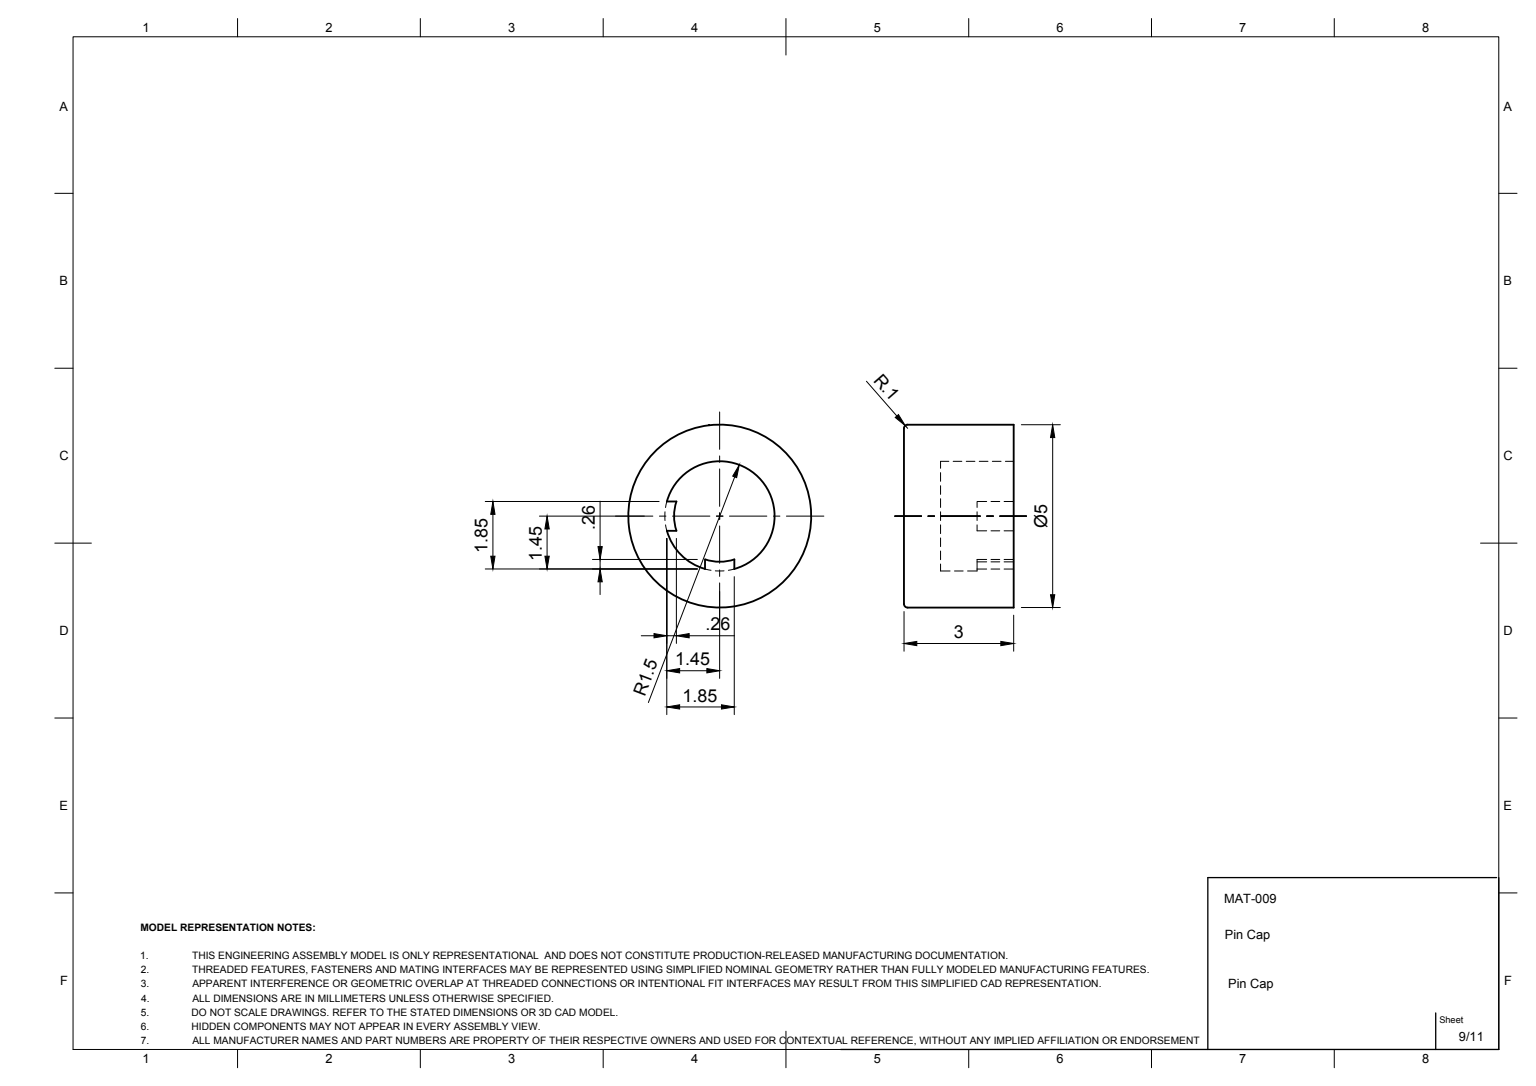
ISO-10303-21;
HEADER;
/* Generated by software containing ST-Developer
 * from STEP Tools, Inc. (www.steptools.com) 
 */

FILE_DESCRIPTION(
/* description */ ('STEP AP214'),
/* implementation_level */ '2;1');

FILE_NAME(
/* name */ 'Pin Cap.step',
/* time_stamp */ '2026-11-14T05:43:09-08:00',
/* author */ (''),
/* organization */ (''),
/* preprocessor_version */ 'ST-DEVELOPER v20.2',
/* originating_system */ 'Autodesk Translation Framework v15.17.0.0',
/* authorisation */ '');

FILE_SCHEMA (('AUTOMOTIVE_DESIGN { 1 0 10303 214 3 1 1 }'));
ENDSEC;

DATA;
#10=MECHANICAL_DESIGN_GEOMETRIC_PRESENTATION_REPRESENTATION('',(#154),#11933);
#127=TOROIDAL_SURFACE('',#7592,2.4,0.1);
#136=SHAPE_REPRESENTATION_RELATIONSHIP('SRR','None',#11996,#145);
#145=ADVANCED_BREP_SHAPE_REPRESENTATION('',(#163),#11932);
#154=STYLED_ITEM('',(#12043),#163);
#163=MANIFOLD_SOLID_BREP('Body1',#6651);
#208=FACE_BOUND('',#1064,.T.);
#310=PLANE('',#7609);
#311=PLANE('',#7611);
#312=PLANE('',#7612);
#313=PLANE('',#7615);
#314=PLANE('',#7616);
#315=PLANE('',#7617);
#316=PLANE('',#7618);
#317=PLANE('',#7619);
#318=PLANE('',#7620);
#659=FACE_OUTER_BOUND('',#1057,.T.);
#660=FACE_OUTER_BOUND('',#1058,.T.);
#661=FACE_OUTER_BOUND('',#1059,.T.);
#662=FACE_OUTER_BOUND('',#1060,.T.);
#663=FACE_OUTER_BOUND('',#1061,.T.);
#664=FACE_OUTER_BOUND('',#1062,.T.);
#665=FACE_OUTER_BOUND('',#1063,.T.);
#666=FACE_OUTER_BOUND('',#1065,.T.);
#667=FACE_OUTER_BOUND('',#1066,.T.);
#668=FACE_OUTER_BOUND('',#1067,.T.);
#669=FACE_OUTER_BOUND('',#1068,.T.);
#670=FACE_OUTER_BOUND('',#1069,.T.);
#671=FACE_OUTER_BOUND('',#1070,.T.);
#672=FACE_OUTER_BOUND('',#1071,.T.);
#1057=EDGE_LOOP('',(#5980,#5981,#5982,#5983,#5984));
#1058=EDGE_LOOP('',(#5985,#5986,#5987,#5988));
#1059=EDGE_LOOP('',(#5989,#5990,#5991,#5992,#5993));
#1060=EDGE_LOOP('',(#5994,#5995,#5996,#5997,#5998,#5999,#6000,#6001,#6002,
#6003,#6004,#6005));
#1061=EDGE_LOOP('',(#6006,#6007,#6008,#6009));
#1062=EDGE_LOOP('',(#6010,#6011,#6012,#6013));
#1063=EDGE_LOOP('',(#6014));
#1064=EDGE_LOOP('',(#6015,#6016,#6017,#6018,#6019,#6020,#6021,#6022,#6023));
#1065=EDGE_LOOP('',(#6024,#6025,#6026,#6027));
#1066=EDGE_LOOP('',(#6028,#6029,#6030,#6031));
#1067=EDGE_LOOP('',(#6032,#6033,#6034,#6035));
#1068=EDGE_LOOP('',(#6036,#6037,#6038,#6039));
#1069=EDGE_LOOP('',(#6040,#6041,#6042,#6043));
#1070=EDGE_LOOP('',(#6044));
#1071=EDGE_LOOP('',(#6045));
#1516=LINE('',#11827,#1978);
#1517=LINE('',#11830,#1979);
#1518=LINE('',#11833,#1980);
#1519=LINE('',#11840,#1981);
#1520=LINE('',#11844,#1982);
#1521=LINE('',#11849,#1983);
#1522=LINE('',#11853,#1984);
#1523=LINE('',#11856,#1985);
#1524=LINE('',#11859,#1986);
#1525=LINE('',#11862,#1987);
#1526=LINE('',#11864,#1988);
#1527=LINE('',#11865,#1989);
#1528=LINE('',#11868,#1990);
#1529=LINE('',#11871,#1991);
#1530=LINE('',#11872,#1992);
#1531=LINE('',#11873,#1993);
#1532=LINE('',#11875,#1994);
#1533=LINE('',#11876,#1995);
#1978=VECTOR('',#9788,1000.);
#1979=VECTOR('',#9791,1000.);
#1980=VECTOR('',#9794,2.5);
#1981=VECTOR('',#9801,1000.);
#1982=VECTOR('',#9804,1.5);
#1983=VECTOR('',#9809,1000.);
#1984=VECTOR('',#9812,1000.);
#1985=VECTOR('',#9815,1000.);
#1986=VECTOR('',#9818,1000.);
#1987=VECTOR('',#9821,1000.);
#1988=VECTOR('',#9824,1000.);
#1989=VECTOR('',#9825,1000.);
#1990=VECTOR('',#9828,1000.);
#1991=VECTOR('',#9831,1000.);
#1992=VECTOR('',#9832,1000.);
#1993=VECTOR('',#9833,1000.);
#1994=VECTOR('',#9836,1000.);
#1995=VECTOR('',#9837,1000.);
#2486=CIRCLE('',#7593,2.5);
#2487=CIRCLE('',#7594,2.5);
#2488=CIRCLE('',#7595,0.1);
#2489=CIRCLE('',#7596,2.4);
#2490=CIRCLE('',#7598,1.25);
#2491=CIRCLE('',#7599,1.25);
#2492=CIRCLE('',#7601,2.5);
#2493=CIRCLE('',#7603,1.5);
#2494=CIRCLE('',#7604,1.5);
#2495=CIRCLE('',#7605,1.5);
#2496=CIRCLE('',#7606,1.5);
#2497=CIRCLE('',#7607,1.5);
#2498=CIRCLE('',#7608,1.5);
#2499=CIRCLE('',#7610,1.25);
#2500=CIRCLE('',#7613,1.25);
#3123=VERTEX_POINT('',#11815);
#3124=VERTEX_POINT('',#11816);
#3125=VERTEX_POINT('',#11819);
#3126=VERTEX_POINT('',#11823);
#3127=VERTEX_POINT('',#11824);
#3128=VERTEX_POINT('',#11826);
#3129=VERTEX_POINT('',#11828);
#3130=VERTEX_POINT('',#11832);
#3131=VERTEX_POINT('',#11836);
#3132=VERTEX_POINT('',#11837);
#3133=VERTEX_POINT('',#11839);
#3134=VERTEX_POINT('',#11841);
#3135=VERTEX_POINT('',#11843);
#3136=VERTEX_POINT('',#11846);
#3137=VERTEX_POINT('',#11848);
#3138=VERTEX_POINT('',#11850);
#3139=VERTEX_POINT('',#11852);
#3140=VERTEX_POINT('',#11854);
#3141=VERTEX_POINT('',#11858);
#3142=VERTEX_POINT('',#11860);
#3143=VERTEX_POINT('',#11867);
#3144=VERTEX_POINT('',#11869);
#4079=EDGE_CURVE('',#3123,#3124,#2486,.T.);
#4080=EDGE_CURVE('',#3124,#3123,#2487,.T.);
#4081=EDGE_CURVE('',#3124,#3125,#2488,.T.);
#4082=EDGE_CURVE('',#3125,#3125,#2489,.T.);
#4083=EDGE_CURVE('',#3126,#3127,#2490,.T.);
#4084=EDGE_CURVE('',#3127,#3128,#1516,.T.);
#4085=EDGE_CURVE('',#3129,#3128,#2491,.T.);
#4086=EDGE_CURVE('',#3126,#3129,#1517,.T.);
#4087=EDGE_CURVE('',#3123,#3130,#1518,.T.);
#4088=EDGE_CURVE('',#3130,#3130,#2492,.T.);
#4089=EDGE_CURVE('',#3131,#3132,#2493,.T.);
#4090=EDGE_CURVE('',#3133,#3132,#1519,.T.);
#4091=EDGE_CURVE('',#3133,#3134,#2494,.T.);
#4092=EDGE_CURVE('',#3134,#3135,#1520,.T.);
#4093=EDGE_CURVE('',#3135,#3135,#2495,.T.);
#4094=EDGE_CURVE('',#3134,#3136,#2496,.T.);
#4095=EDGE_CURVE('',#3136,#3137,#1521,.T.);
#4096=EDGE_CURVE('',#3137,#3138,#2497,.T.);
#4097=EDGE_CURVE('',#3139,#3138,#1522,.T.);
#4098=EDGE_CURVE('',#3139,#3140,#2498,.T.);
#4099=EDGE_CURVE('',#3140,#3131,#1523,.T.);
#4100=EDGE_CURVE('',#3137,#3141,#1524,.T.);
#4101=EDGE_CURVE('',#3141,#3142,#2499,.T.);
#4102=EDGE_CURVE('',#3142,#3138,#1525,.T.);
#4103=EDGE_CURVE('',#3131,#3129,#1526,.T.);
#4104=EDGE_CURVE('',#3128,#3132,#1527,.T.);
#4105=EDGE_CURVE('',#3143,#3139,#1528,.T.);
#4106=EDGE_CURVE('',#3144,#3143,#2500,.T.);
#4107=EDGE_CURVE('',#3136,#3144,#1529,.T.);
#4108=EDGE_CURVE('',#3127,#3133,#1530,.T.);
#4109=EDGE_CURVE('',#3140,#3126,#1531,.T.);
#4110=EDGE_CURVE('',#3144,#3141,#1532,.T.);
#4111=EDGE_CURVE('',#3143,#3142,#1533,.T.);
#5980=ORIENTED_EDGE('',*,*,#4079,.F.);
#5981=ORIENTED_EDGE('',*,*,#4080,.F.);
#5982=ORIENTED_EDGE('',*,*,#4081,.T.);
#5983=ORIENTED_EDGE('',*,*,#4082,.F.);
#5984=ORIENTED_EDGE('',*,*,#4081,.F.);
#5985=ORIENTED_EDGE('',*,*,#4083,.T.);
#5986=ORIENTED_EDGE('',*,*,#4084,.T.);
#5987=ORIENTED_EDGE('',*,*,#4085,.F.);
#5988=ORIENTED_EDGE('',*,*,#4086,.F.);
#5989=ORIENTED_EDGE('',*,*,#4079,.T.);
#5990=ORIENTED_EDGE('',*,*,#4080,.T.);
#5991=ORIENTED_EDGE('',*,*,#4087,.T.);
#5992=ORIENTED_EDGE('',*,*,#4088,.F.);
#5993=ORIENTED_EDGE('',*,*,#4087,.F.);
#5994=ORIENTED_EDGE('',*,*,#4089,.T.);
#5995=ORIENTED_EDGE('',*,*,#4090,.F.);
#5996=ORIENTED_EDGE('',*,*,#4091,.T.);
#5997=ORIENTED_EDGE('',*,*,#4092,.T.);
#5998=ORIENTED_EDGE('',*,*,#4093,.T.);
#5999=ORIENTED_EDGE('',*,*,#4092,.F.);
#6000=ORIENTED_EDGE('',*,*,#4094,.T.);
#6001=ORIENTED_EDGE('',*,*,#4095,.T.);
#6002=ORIENTED_EDGE('',*,*,#4096,.T.);
#6003=ORIENTED_EDGE('',*,*,#4097,.F.);
#6004=ORIENTED_EDGE('',*,*,#4098,.T.);
#6005=ORIENTED_EDGE('',*,*,#4099,.T.);
#6006=ORIENTED_EDGE('',*,*,#4096,.F.);
#6007=ORIENTED_EDGE('',*,*,#4100,.T.);
#6008=ORIENTED_EDGE('',*,*,#4101,.T.);
#6009=ORIENTED_EDGE('',*,*,#4102,.T.);
#6010=ORIENTED_EDGE('',*,*,#4089,.F.);
#6011=ORIENTED_EDGE('',*,*,#4103,.T.);
#6012=ORIENTED_EDGE('',*,*,#4085,.T.);
#6013=ORIENTED_EDGE('',*,*,#4104,.T.);
#6014=ORIENTED_EDGE('',*,*,#4088,.T.);
#6015=ORIENTED_EDGE('',*,*,#4105,.F.);
#6016=ORIENTED_EDGE('',*,*,#4106,.F.);
#6017=ORIENTED_EDGE('',*,*,#4107,.F.);
#6018=ORIENTED_EDGE('',*,*,#4094,.F.);
#6019=ORIENTED_EDGE('',*,*,#4091,.F.);
#6020=ORIENTED_EDGE('',*,*,#4108,.F.);
#6021=ORIENTED_EDGE('',*,*,#4083,.F.);
#6022=ORIENTED_EDGE('',*,*,#4109,.F.);
#6023=ORIENTED_EDGE('',*,*,#4098,.F.);
#6024=ORIENTED_EDGE('',*,*,#4101,.F.);
#6025=ORIENTED_EDGE('',*,*,#4110,.F.);
#6026=ORIENTED_EDGE('',*,*,#4106,.T.);
#6027=ORIENTED_EDGE('',*,*,#4111,.T.);
#6028=ORIENTED_EDGE('',*,*,#4102,.F.);
#6029=ORIENTED_EDGE('',*,*,#4111,.F.);
#6030=ORIENTED_EDGE('',*,*,#4105,.T.);
#6031=ORIENTED_EDGE('',*,*,#4097,.T.);
#6032=ORIENTED_EDGE('',*,*,#4103,.F.);
#6033=ORIENTED_EDGE('',*,*,#4099,.F.);
#6034=ORIENTED_EDGE('',*,*,#4109,.T.);
#6035=ORIENTED_EDGE('',*,*,#4086,.T.);
#6036=ORIENTED_EDGE('',*,*,#4104,.F.);
#6037=ORIENTED_EDGE('',*,*,#4084,.F.);
#6038=ORIENTED_EDGE('',*,*,#4108,.T.);
#6039=ORIENTED_EDGE('',*,*,#4090,.T.);
#6040=ORIENTED_EDGE('',*,*,#4100,.F.);
#6041=ORIENTED_EDGE('',*,*,#4095,.F.);
#6042=ORIENTED_EDGE('',*,*,#4107,.T.);
#6043=ORIENTED_EDGE('',*,*,#4110,.T.);
#6044=ORIENTED_EDGE('',*,*,#4082,.T.);
#6045=ORIENTED_EDGE('',*,*,#4093,.F.);
#6285=CYLINDRICAL_SURFACE('',#7597,1.25);
#6286=CYLINDRICAL_SURFACE('',#7600,2.5);
#6287=CYLINDRICAL_SURFACE('',#7602,1.5);
#6288=CYLINDRICAL_SURFACE('',#7614,1.25);
#6629=ADVANCED_FACE('',(#659),#127,.T.);
#6630=ADVANCED_FACE('',(#660),#6285,.F.);
#6631=ADVANCED_FACE('',(#661),#6286,.T.);
#6632=ADVANCED_FACE('',(#662),#6287,.F.);
#6633=ADVANCED_FACE('',(#663),#310,.F.);
#6634=ADVANCED_FACE('',(#664),#311,.F.);
#6635=ADVANCED_FACE('',(#665,#208),#312,.T.);
#6636=ADVANCED_FACE('',(#666),#6288,.F.);
#6637=ADVANCED_FACE('',(#667),#313,.T.);
#6638=ADVANCED_FACE('',(#668),#314,.T.);
#6639=ADVANCED_FACE('',(#669),#315,.T.);
#6640=ADVANCED_FACE('',(#670),#316,.T.);
#6641=ADVANCED_FACE('',(#671),#317,.F.);
#6642=ADVANCED_FACE('',(#672),#318,.F.);
#6651=CLOSED_SHELL('',(#6629,#6630,#6631,#6632,#6633,#6634,#6635,#6636,
#6637,#6638,#6639,#6640,#6641,#6642));
#7591=AXIS2_PLACEMENT_3D('',#11813,#9772,#9773);
#7592=AXIS2_PLACEMENT_3D('',#11814,#9774,#9775);
#7593=AXIS2_PLACEMENT_3D('',#11817,#9776,#9777);
#7594=AXIS2_PLACEMENT_3D('',#11818,#9778,#9779);
#7595=AXIS2_PLACEMENT_3D('',#11820,#9780,#9781);
#7596=AXIS2_PLACEMENT_3D('',#11821,#9782,#9783);
#7597=AXIS2_PLACEMENT_3D('',#11822,#9784,#9785);
#7598=AXIS2_PLACEMENT_3D('',#11825,#9786,#9787);
#7599=AXIS2_PLACEMENT_3D('',#11829,#9789,#9790);
#7600=AXIS2_PLACEMENT_3D('',#11831,#9792,#9793);
#7601=AXIS2_PLACEMENT_3D('',#11834,#9795,#9796);
#7602=AXIS2_PLACEMENT_3D('',#11835,#9797,#9798);
#7603=AXIS2_PLACEMENT_3D('',#11838,#9799,#9800);
#7604=AXIS2_PLACEMENT_3D('',#11842,#9802,#9803);
#7605=AXIS2_PLACEMENT_3D('',#11845,#9805,#9806);
#7606=AXIS2_PLACEMENT_3D('',#11847,#9807,#9808);
#7607=AXIS2_PLACEMENT_3D('',#11851,#9810,#9811);
#7608=AXIS2_PLACEMENT_3D('',#11855,#9813,#9814);
#7609=AXIS2_PLACEMENT_3D('',#11857,#9816,#9817);
#7610=AXIS2_PLACEMENT_3D('',#11861,#9819,#9820);
#7611=AXIS2_PLACEMENT_3D('',#11863,#9822,#9823);
#7612=AXIS2_PLACEMENT_3D('',#11866,#9826,#9827);
#7613=AXIS2_PLACEMENT_3D('',#11870,#9829,#9830);
#7614=AXIS2_PLACEMENT_3D('',#11874,#9834,#9835);
#7615=AXIS2_PLACEMENT_3D('',#11877,#9838,#9839);
#7616=AXIS2_PLACEMENT_3D('',#11878,#9840,#9841);
#7617=AXIS2_PLACEMENT_3D('',#11879,#9842,#9843);
#7618=AXIS2_PLACEMENT_3D('',#11880,#9844,#9845);
#7619=AXIS2_PLACEMENT_3D('',#11881,#9846,#9847);
#7620=AXIS2_PLACEMENT_3D('',#11882,#9848,#9849);
#9772=DIRECTION('axis',(0.,0.,1.));
#9773=DIRECTION('refdir',(1.,0.,0.));
#9774=DIRECTION('center_axis',(0.,0.,1.));
#9775=DIRECTION('ref_axis',(1.,0.,0.));
#9776=DIRECTION('center_axis',(0.,0.,1.));
#9777=DIRECTION('ref_axis',(1.,0.,0.));
#9778=DIRECTION('center_axis',(0.,0.,1.));
#9779=DIRECTION('ref_axis',(1.,0.,0.));
#9780=DIRECTION('center_axis',(1.22464679914735E-16,-1.,0.));
#9781=DIRECTION('ref_axis',(-1.,-1.22464679914735E-16,0.));
#9782=DIRECTION('center_axis',(0.,0.,-1.));
#9783=DIRECTION('ref_axis',(1.,0.,0.));
#9784=DIRECTION('center_axis',(0.,0.,-1.));
#9785=DIRECTION('ref_axis',(-1.,0.,0.));
#9786=DIRECTION('center_axis',(0.,0.,1.));
#9787=DIRECTION('ref_axis',(1.,0.,0.));
#9788=DIRECTION('',(0.,0.,-1.));
#9789=DIRECTION('center_axis',(0.,0.,1.));
#9790=DIRECTION('ref_axis',(1.,0.,0.));
#9791=DIRECTION('',(0.,0.,-1.));
#9792=DIRECTION('center_axis',(0.,0.,-1.));
#9793=DIRECTION('ref_axis',(-1.,0.,0.));
#9794=DIRECTION('',(0.,0.,1.));
#9795=DIRECTION('center_axis',(0.,0.,1.));
#9796=DIRECTION('ref_axis',(1.,0.,0.));
#9797=DIRECTION('center_axis',(0.,0.,-1.));
#9798=DIRECTION('ref_axis',(-1.,0.,0.));
#9799=DIRECTION('center_axis',(0.,0.,1.));
#9800=DIRECTION('ref_axis',(1.,0.,0.));
#9801=DIRECTION('',(0.,0.,-1.));
#9802=DIRECTION('center_axis',(0.,0.,1.));
#9803=DIRECTION('ref_axis',(1.,0.,0.));
#9804=DIRECTION('',(0.,0.,-1.));
#9805=DIRECTION('center_axis',(0.,0.,-1.));
#9806=DIRECTION('ref_axis',(-1.,0.,0.));
#9807=DIRECTION('center_axis',(0.,0.,1.));
#9808=DIRECTION('ref_axis',(1.,0.,0.));
#9809=DIRECTION('',(0.,0.,-1.));
#9810=DIRECTION('center_axis',(0.,0.,1.));
#9811=DIRECTION('ref_axis',(1.,0.,0.));
#9812=DIRECTION('',(0.,0.,-1.));
#9813=DIRECTION('center_axis',(0.,0.,1.));
#9814=DIRECTION('ref_axis',(1.,0.,0.));
#9815=DIRECTION('',(0.,0.,-1.));
#9816=DIRECTION('center_axis',(0.,0.,1.));
#9817=DIRECTION('ref_axis',(1.,0.,0.));
#9818=DIRECTION('',(-2.07374770584121E-16,-1.,0.));
#9819=DIRECTION('center_axis',(0.,0.,1.));
#9820=DIRECTION('ref_axis',(1.,0.,0.));
#9821=DIRECTION('',(-2.07374770584121E-16,1.,0.));
#9822=DIRECTION('center_axis',(0.,0.,1.));
#9823=DIRECTION('ref_axis',(1.,0.,0.));
#9824=DIRECTION('',(1.,0.,0.));
#9825=DIRECTION('',(-1.,0.,0.));
#9826=DIRECTION('center_axis',(0.,0.,1.));
#9827=DIRECTION('ref_axis',(1.,0.,0.));
#9828=DIRECTION('',(-2.07374770584121E-16,1.,0.));
#9829=DIRECTION('center_axis',(0.,0.,1.));
#9830=DIRECTION('ref_axis',(1.,0.,0.));
#9831=DIRECTION('',(-2.07374770584121E-16,-1.,0.));
#9832=DIRECTION('',(-1.,0.,0.));
#9833=DIRECTION('',(1.,0.,0.));
#9834=DIRECTION('center_axis',(0.,0.,-1.));
#9835=DIRECTION('ref_axis',(-1.,0.,0.));
#9836=DIRECTION('',(0.,0.,-1.));
#9837=DIRECTION('',(0.,0.,-1.));
#9838=DIRECTION('center_axis',(-1.,-2.07374770584121E-16,0.));
#9839=DIRECTION('ref_axis',(2.07374770584121E-16,-1.,0.));
#9840=DIRECTION('center_axis',(0.,1.,0.));
#9841=DIRECTION('ref_axis',(0.,0.,1.));
#9842=DIRECTION('center_axis',(0.,-1.,0.));
#9843=DIRECTION('ref_axis',(0.,0.,-1.));
#9844=DIRECTION('center_axis',(1.,-2.07374770584121E-16,0.));
#9845=DIRECTION('ref_axis',(2.07374770584121E-16,1.,0.));
#9846=DIRECTION('center_axis',(0.,0.,1.));
#9847=DIRECTION('ref_axis',(1.,0.,0.));
#9848=DIRECTION('center_axis',(0.,0.,-1.));
#9849=DIRECTION('ref_axis',(-1.,0.,0.));
#11813=CARTESIAN_POINT('',(0.,0.,0.));
#11814=CARTESIAN_POINT('Origin',(0.,0.,-1.9));
#11815=CARTESIAN_POINT('',(2.5,3.06161699786838E-16,-1.9));
#11816=CARTESIAN_POINT('',(-2.5,-3.06161699786838E-16,-1.9));
#11817=CARTESIAN_POINT('Origin',(0.,0.,-1.9));
#11818=CARTESIAN_POINT('Origin',(0.,0.,-1.9));
#11819=CARTESIAN_POINT('',(-2.4,-2.93915231795365E-16,-2.));
#11820=CARTESIAN_POINT('Origin',(-2.4,-2.93915231795365E-16,-1.9));
#11821=CARTESIAN_POINT('Origin',(0.,0.,-2.));
#11822=CARTESIAN_POINT('Origin',(0.,0.,1.));
#11823=CARTESIAN_POINT('',(-1.1842719282327,0.4,1.));
#11824=CARTESIAN_POINT('',(-1.1842719282327,-0.4,1.));
#11825=CARTESIAN_POINT('Origin',(0.,0.,1.));
#11826=CARTESIAN_POINT('',(-1.1842719282327,-0.4,0.));
#11827=CARTESIAN_POINT('',(-1.1842719282327,-0.4,1.));
#11828=CARTESIAN_POINT('',(-1.1842719282327,0.4,0.));
#11829=CARTESIAN_POINT('Origin',(0.,0.,0.));
#11830=CARTESIAN_POINT('',(-1.1842719282327,0.4,1.));
#11831=CARTESIAN_POINT('Origin',(0.,0.,1.));
#11832=CARTESIAN_POINT('',(2.5,-3.06161699786838E-16,1.));
#11833=CARTESIAN_POINT('',(2.5,-3.06161699786838E-16,1.));
#11834=CARTESIAN_POINT('Origin',(0.,0.,1.));
#11835=CARTESIAN_POINT('Origin',(0.,0.,1.));
#11836=CARTESIAN_POINT('',(-1.4456832294801,0.4,0.));
#11837=CARTESIAN_POINT('',(-1.4456832294801,-0.4,0.));
#11838=CARTESIAN_POINT('Origin',(0.,0.,0.));
#11839=CARTESIAN_POINT('',(-1.4456832294801,-0.4,1.));
#11840=CARTESIAN_POINT('',(-1.4456832294801,-0.4,1.));
#11841=CARTESIAN_POINT('',(1.5,-1.83697019872103E-16,1.));
#11842=CARTESIAN_POINT('Origin',(0.,0.,1.));
#11843=CARTESIAN_POINT('',(1.5,-1.83697019872103E-16,-1.));
#11844=CARTESIAN_POINT('',(1.5,-1.83697019872103E-16,1.));
#11845=CARTESIAN_POINT('Origin',(0.,0.,-1.));
#11846=CARTESIAN_POINT('',(0.4,1.4456832294801,1.));
#11847=CARTESIAN_POINT('Origin',(0.,0.,1.));
#11848=CARTESIAN_POINT('',(0.4,1.4456832294801,0.));
#11849=CARTESIAN_POINT('',(0.4,1.4456832294801,1.));
#11850=CARTESIAN_POINT('',(-0.4,1.4456832294801,0.));
#11851=CARTESIAN_POINT('Origin',(0.,0.,0.));
#11852=CARTESIAN_POINT('',(-0.4,1.4456832294801,1.));
#11853=CARTESIAN_POINT('',(-0.4,1.4456832294801,1.));
#11854=CARTESIAN_POINT('',(-1.4456832294801,0.4,1.));
#11855=CARTESIAN_POINT('Origin',(0.,0.,1.));
#11856=CARTESIAN_POINT('',(-1.4456832294801,0.4,1.));
#11857=CARTESIAN_POINT('Origin',(0.,0.,0.));
#11858=CARTESIAN_POINT('',(0.4,1.1842719282327,0.));
#11859=CARTESIAN_POINT('',(0.4,1.1842719282327,0.));
#11860=CARTESIAN_POINT('',(-0.4,1.1842719282327,0.));
#11861=CARTESIAN_POINT('Origin',(0.,0.,0.));
#11862=CARTESIAN_POINT('',(-0.4,1.1842719282327,0.));
#11863=CARTESIAN_POINT('Origin',(0.,0.,0.));
#11864=CARTESIAN_POINT('',(-1.1842719282327,0.4,0.));
#11865=CARTESIAN_POINT('',(-1.1842719282327,-0.4,0.));
#11866=CARTESIAN_POINT('Origin',(0.,0.,1.));
#11867=CARTESIAN_POINT('',(-0.4,1.1842719282327,1.));
#11868=CARTESIAN_POINT('',(-0.4,1.1842719282327,1.));
#11869=CARTESIAN_POINT('',(0.4,1.1842719282327,1.));
#11870=CARTESIAN_POINT('Origin',(0.,0.,1.));
#11871=CARTESIAN_POINT('',(0.4,1.1842719282327,1.));
#11872=CARTESIAN_POINT('',(-1.1842719282327,-0.4,1.));
#11873=CARTESIAN_POINT('',(-1.1842719282327,0.4,1.));
#11874=CARTESIAN_POINT('Origin',(0.,0.,1.));
#11875=CARTESIAN_POINT('',(0.4,1.1842719282327,1.));
#11876=CARTESIAN_POINT('',(-0.4,1.1842719282327,1.));
#11877=CARTESIAN_POINT('Origin',(-0.4,1.1842719282327,1.));
#11878=CARTESIAN_POINT('Origin',(-1.1842719282327,0.4,1.));
#11879=CARTESIAN_POINT('Origin',(-1.1842719282327,-0.4,1.));
#11880=CARTESIAN_POINT('Origin',(0.4,1.1842719282327,1.));
#11881=CARTESIAN_POINT('Origin',(0.,0.,-2.));
#11882=CARTESIAN_POINT('Origin',(0.,0.,-1.));
#11921=UNCERTAINTY_MEASURE_WITH_UNIT(LENGTH_MEASURE(0.01),#11934,
'DISTANCE_ACCURACY_VALUE',
'Maximum model space distance between geometric entities at asserted c
onnectivities');
#11922=UNCERTAINTY_MEASURE_WITH_UNIT(LENGTH_MEASURE(0.01),#11934,
'DISTANCE_ACCURACY_VALUE',
'Maximum model space distance between geometric entities at asserted c
onnectivities');
#11932=(
GEOMETRIC_REPRESENTATION_CONTEXT(3)
GLOBAL_UNCERTAINTY_ASSIGNED_CONTEXT((#11921))
GLOBAL_UNIT_ASSIGNED_CONTEXT((#11934,#11936,#11937))
REPRESENTATION_CONTEXT('','3D')
);
#11933=(
GEOMETRIC_REPRESENTATION_CONTEXT(3)
GLOBAL_UNCERTAINTY_ASSIGNED_CONTEXT((#11922))
GLOBAL_UNIT_ASSIGNED_CONTEXT((#11934,#11936,#11937))
REPRESENTATION_CONTEXT('','3D')
);
#11934=(
LENGTH_UNIT()
NAMED_UNIT(*)
SI_UNIT(.MILLI.,.METRE.)
);
#11936=(
NAMED_UNIT(*)
PLANE_ANGLE_UNIT()
SI_UNIT($,.RADIAN.)
);
#11937=(
NAMED_UNIT(*)
SI_UNIT($,.STERADIAN.)
SOLID_ANGLE_UNIT()
);
#11947=SHAPE_DEFINITION_REPRESENTATION(#11957,#11996);
#11957=PRODUCT_DEFINITION_SHAPE('',$,#12007);
#11996=SHAPE_REPRESENTATION('',(#7591),#11932);
#11997=PRODUCT_DEFINITION_CONTEXT('part definition',#12029,'design');
#12007=PRODUCT_DEFINITION('Pin Cap','Pin Cap',#12017,#11997);
#12017=PRODUCT_DEFINITION_FORMATION('',$,#12040);
#12029=APPLICATION_CONTEXT(
'Core Data for Automotive Mechanical Design Process');
#12030=PRODUCT_CONTEXT('part definition',#12029,'mechanical');
#12040=PRODUCT('Pin Cap','Pin Cap',$,(#12030));
#12043=PRESENTATION_STYLE_ASSIGNMENT((#12047));
#12047=SURFACE_STYLE_USAGE(.BOTH.,#12051);
#12051=SURFACE_SIDE_STYLE('',(#12055));
#12055=SURFACE_STYLE_FILL_AREA(#12059);
#12059=FILL_AREA_STYLE('Opaque(61,176,222)',(#12063));
#12063=FILL_AREA_STYLE_COLOUR('Opaque(61,176,222)',#12067);
#12067=COLOUR_RGB('Opaque(61,176,222)',0.23921568627451,0.690196078431373,
0.870588235294118);
ENDSEC;
END-ISO-10303-21;
